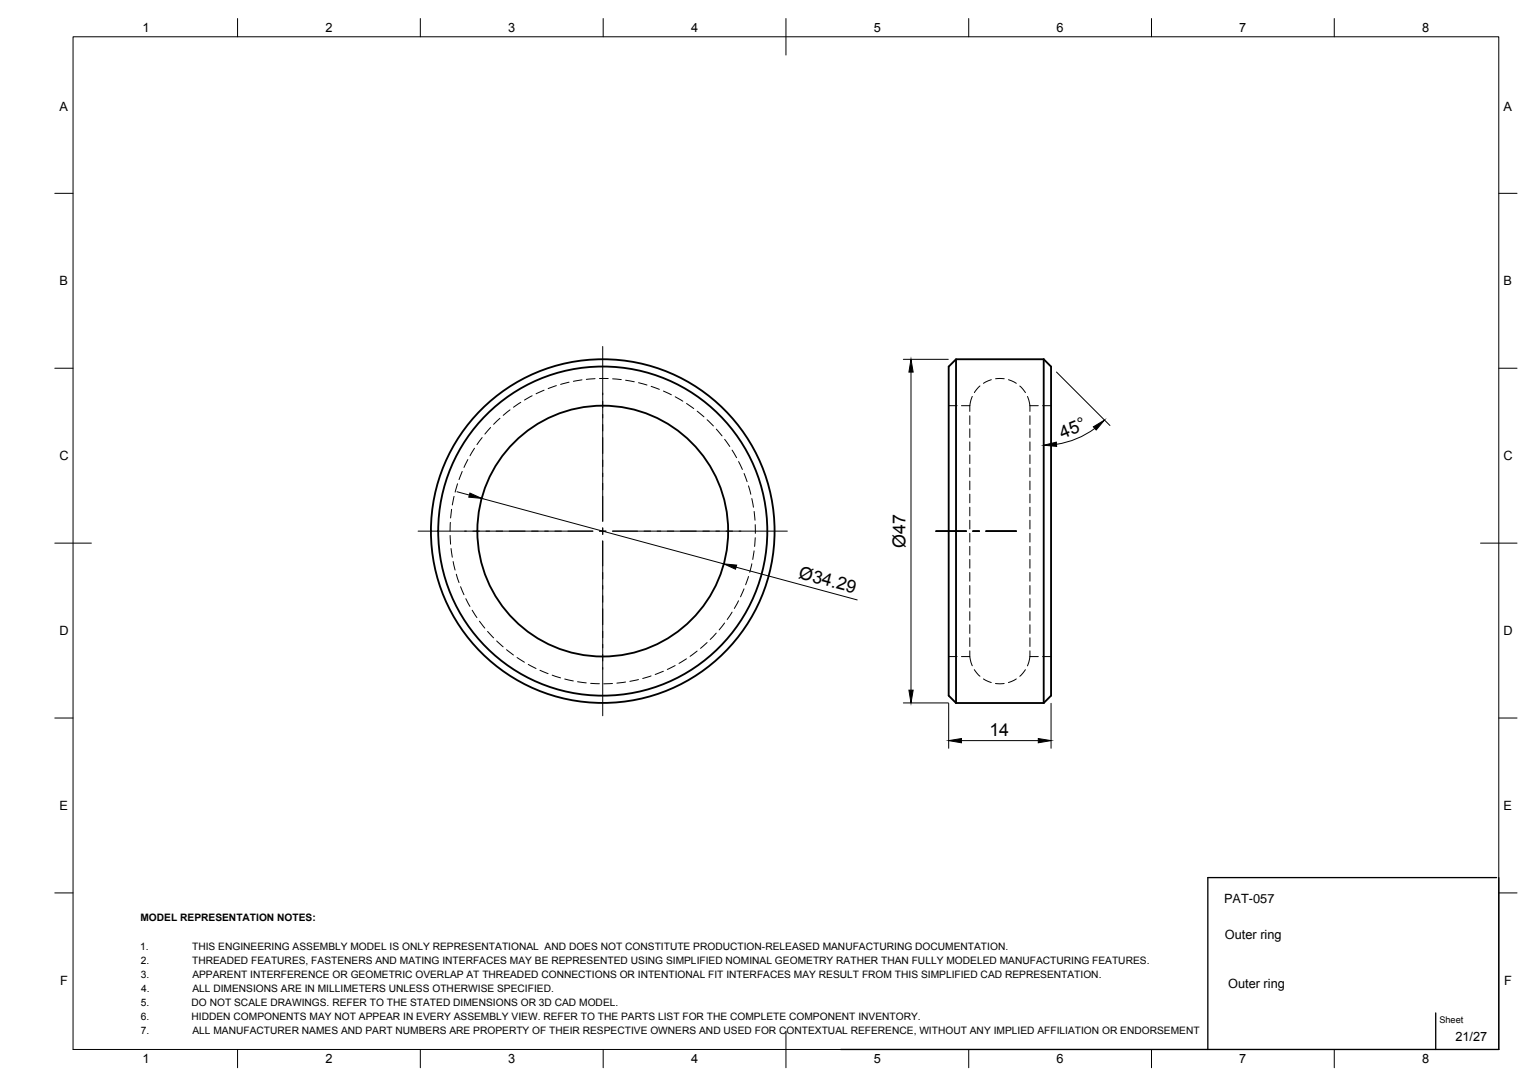
ISO-10303-21;
HEADER;
/* Generated by software containing ST-Developer
 * from STEP Tools, Inc. (www.steptools.com) 
 */

FILE_DESCRIPTION(
/* description */ ('Bearing-mounted hook block'),
/* implementation_level */ '2;1');

FILE_NAME(
/* name */ 'Outer ring.step',
/* time_stamp */ '2026-10-28T22:30:11-07:00',
/* author */ (''),
/* organization */ (''),
/* preprocessor_version */ 'ST-DEVELOPER v20.2',
/* originating_system */ 'Autodesk Translation Framework v15.17.0.0',
/* authorisation */ '');

FILE_SCHEMA (('AUTOMOTIVE_DESIGN { 1 0 10303 214 3 1 1 }'));
ENDSEC;

DATA;
#10=MECHANICAL_DESIGN_GEOMETRIC_PRESENTATION_REPRESENTATION('',(#338),#7609);
#46=TOROIDAL_SURFACE('',#4525,1.675,0.412776);
#264=CONICAL_SURFACE('',#4536,2.3,0.785398163397449);
#265=CONICAL_SURFACE('',#4540,2.3,0.785398163397449);
#290=SHAPE_REPRESENTATION_RELATIONSHIP('SRR','None',#7739,#314);
#314=ADVANCED_BREP_SHAPE_REPRESENTATION('',(#368),#7599);
#338=STYLED_ITEM('',(#7931),#368);
#368=MANIFOLD_SOLID_BREP('Body1',#3936);
#530=LINE('',#6748,#760);
#531=LINE('',#6757,#761);
#532=LINE('',#6761,#762);
#533=LINE('',#6765,#763);
#534=LINE('',#6768,#764);
#760=VECTOR('',#5531,1.71469);
#761=VECTOR('',#5542,2.3);
#762=VECTOR('',#5547,2.35);
#763=VECTOR('',#5552,2.3);
#764=VECTOR('',#5557,1.71469);
#895=CYLINDRICAL_SURFACE('',#4531,1.71469);
#896=CYLINDRICAL_SURFACE('',#4538,2.35);
#897=CYLINDRICAL_SURFACE('',#4543,1.71469);
#976=FACE_BOUND('',#1433,.T.);
#977=FACE_BOUND('',#1438,.T.);
#1139=FACE_OUTER_BOUND('',#1430,.T.);
#1140=FACE_OUTER_BOUND('',#1431,.T.);
#1141=FACE_OUTER_BOUND('',#1432,.T.);
#1142=FACE_OUTER_BOUND('',#1434,.T.);
#1143=FACE_OUTER_BOUND('',#1435,.T.);
#1144=FACE_OUTER_BOUND('',#1436,.T.);
#1145=FACE_OUTER_BOUND('',#1437,.T.);
#1146=FACE_OUTER_BOUND('',#1439,.T.);
#1430=EDGE_LOOP('',(#3156,#3157,#3158,#3159,#3160,#3161));
#1431=EDGE_LOOP('',(#3162,#3163,#3164,#3165,#3166));
#1432=EDGE_LOOP('',(#3167));
#1433=EDGE_LOOP('',(#3168));
#1434=EDGE_LOOP('',(#3169,#3170,#3171,#3172));
#1435=EDGE_LOOP('',(#3173,#3174,#3175,#3176));
#1436=EDGE_LOOP('',(#3177,#3178,#3179,#3180));
#1437=EDGE_LOOP('',(#3181));
#1438=EDGE_LOOP('',(#3182));
#1439=EDGE_LOOP('',(#3183,#3184,#3185,#3186,#3187));
#1678=CIRCLE('',#4526,1.71469);
#1679=CIRCLE('',#4527,1.71469);
#1680=CIRCLE('',#4528,0.412776);
#1681=CIRCLE('',#4529,1.71469);
#1682=CIRCLE('',#4530,1.71469);
#1683=CIRCLE('',#4532,1.71469);
#1684=CIRCLE('',#4534,2.25);
#1685=CIRCLE('',#4535,1.71469);
#1686=CIRCLE('',#4537,2.35);
#1687=CIRCLE('',#4539,2.35);
#1688=CIRCLE('',#4541,2.25);
#1962=VERTEX_POINT('',#6736);
#1963=VERTEX_POINT('',#6737);
#1964=VERTEX_POINT('',#6740);
#1965=VERTEX_POINT('',#6742);
#1966=VERTEX_POINT('',#6746);
#1967=VERTEX_POINT('',#6750);
#1968=VERTEX_POINT('',#6752);
#1969=VERTEX_POINT('',#6755);
#1970=VERTEX_POINT('',#6759);
#1971=VERTEX_POINT('',#6763);
#2388=EDGE_CURVE('',#1962,#1963,#1678,.T.);
#2389=EDGE_CURVE('',#1963,#1962,#1679,.T.);
#2390=EDGE_CURVE('',#1963,#1964,#1680,.T.);
#2391=EDGE_CURVE('',#1965,#1964,#1681,.T.);
#2392=EDGE_CURVE('',#1964,#1965,#1682,.T.);
#2393=EDGE_CURVE('',#1966,#1966,#1683,.T.);
#2394=EDGE_CURVE('',#1966,#1965,#530,.T.);
#2395=EDGE_CURVE('',#1967,#1967,#1684,.T.);
#2396=EDGE_CURVE('',#1968,#1968,#1685,.T.);
#2397=EDGE_CURVE('',#1969,#1969,#1686,.T.);
#2398=EDGE_CURVE('',#1969,#1967,#531,.T.);
#2399=EDGE_CURVE('',#1970,#1970,#1687,.T.);
#2400=EDGE_CURVE('',#1970,#1969,#532,.T.);
#2401=EDGE_CURVE('',#1971,#1971,#1688,.T.);
#2402=EDGE_CURVE('',#1971,#1970,#533,.T.);
#2403=EDGE_CURVE('',#1962,#1968,#534,.T.);
#3156=ORIENTED_EDGE('',*,*,#2388,.F.);
#3157=ORIENTED_EDGE('',*,*,#2389,.F.);
#3158=ORIENTED_EDGE('',*,*,#2390,.T.);
#3159=ORIENTED_EDGE('',*,*,#2391,.F.);
#3160=ORIENTED_EDGE('',*,*,#2392,.F.);
#3161=ORIENTED_EDGE('',*,*,#2390,.F.);
#3162=ORIENTED_EDGE('',*,*,#2393,.T.);
#3163=ORIENTED_EDGE('',*,*,#2394,.T.);
#3164=ORIENTED_EDGE('',*,*,#2391,.T.);
#3165=ORIENTED_EDGE('',*,*,#2392,.T.);
#3166=ORIENTED_EDGE('',*,*,#2394,.F.);
#3167=ORIENTED_EDGE('',*,*,#2395,.F.);
#3168=ORIENTED_EDGE('',*,*,#2396,.T.);
#3169=ORIENTED_EDGE('',*,*,#2397,.F.);
#3170=ORIENTED_EDGE('',*,*,#2398,.T.);
#3171=ORIENTED_EDGE('',*,*,#2395,.T.);
#3172=ORIENTED_EDGE('',*,*,#2398,.F.);
#3173=ORIENTED_EDGE('',*,*,#2399,.F.);
#3174=ORIENTED_EDGE('',*,*,#2400,.T.);
#3175=ORIENTED_EDGE('',*,*,#2397,.T.);
#3176=ORIENTED_EDGE('',*,*,#2400,.F.);
#3177=ORIENTED_EDGE('',*,*,#2401,.F.);
#3178=ORIENTED_EDGE('',*,*,#2402,.T.);
#3179=ORIENTED_EDGE('',*,*,#2399,.T.);
#3180=ORIENTED_EDGE('',*,*,#2402,.F.);
#3181=ORIENTED_EDGE('',*,*,#2401,.T.);
#3182=ORIENTED_EDGE('',*,*,#2393,.F.);
#3183=ORIENTED_EDGE('',*,*,#2388,.T.);
#3184=ORIENTED_EDGE('',*,*,#2389,.T.);
#3185=ORIENTED_EDGE('',*,*,#2403,.T.);
#3186=ORIENTED_EDGE('',*,*,#2396,.F.);
#3187=ORIENTED_EDGE('',*,*,#2403,.F.);
#3633=PLANE('',#4533);
#3634=PLANE('',#4542);
#3821=ADVANCED_FACE('',(#1139),#46,.F.);
#3822=ADVANCED_FACE('',(#1140),#895,.F.);
#3823=ADVANCED_FACE('',(#1141,#976),#3633,.T.);
#3824=ADVANCED_FACE('',(#1142),#264,.T.);
#3825=ADVANCED_FACE('',(#1143),#896,.T.);
#3826=ADVANCED_FACE('',(#1144),#265,.T.);
#3827=ADVANCED_FACE('',(#1145,#977),#3634,.T.);
#3828=ADVANCED_FACE('',(#1146),#897,.F.);
#3936=CLOSED_SHELL('',(#3821,#3822,#3823,#3824,#3825,#3826,#3827,#3828));
#4524=AXIS2_PLACEMENT_3D('',#6734,#5513,#5514);
#4525=AXIS2_PLACEMENT_3D('',#6735,#5515,#5516);
#4526=AXIS2_PLACEMENT_3D('',#6738,#5517,#5518);
#4527=AXIS2_PLACEMENT_3D('',#6739,#5519,#5520);
#4528=AXIS2_PLACEMENT_3D('',#6741,#5521,#5522);
#4529=AXIS2_PLACEMENT_3D('',#6743,#5523,#5524);
#4530=AXIS2_PLACEMENT_3D('',#6744,#5525,#5526);
#4531=AXIS2_PLACEMENT_3D('',#6745,#5527,#5528);
#4532=AXIS2_PLACEMENT_3D('',#6747,#5529,#5530);
#4533=AXIS2_PLACEMENT_3D('',#6749,#5532,#5533);
#4534=AXIS2_PLACEMENT_3D('',#6751,#5534,#5535);
#4535=AXIS2_PLACEMENT_3D('',#6753,#5536,#5537);
#4536=AXIS2_PLACEMENT_3D('',#6754,#5538,#5539);
#4537=AXIS2_PLACEMENT_3D('',#6756,#5540,#5541);
#4538=AXIS2_PLACEMENT_3D('',#6758,#5543,#5544);
#4539=AXIS2_PLACEMENT_3D('',#6760,#5545,#5546);
#4540=AXIS2_PLACEMENT_3D('',#6762,#5548,#5549);
#4541=AXIS2_PLACEMENT_3D('',#6764,#5550,#5551);
#4542=AXIS2_PLACEMENT_3D('',#6766,#5553,#5554);
#4543=AXIS2_PLACEMENT_3D('',#6767,#5555,#5556);
#5513=DIRECTION('axis',(0.,0.,1.));
#5514=DIRECTION('refdir',(1.,0.,0.));
#5515=DIRECTION('center_axis',(0.,-1.,0.));
#5516=DIRECTION('ref_axis',(0.,0.,-1.));
#5517=DIRECTION('center_axis',(0.,-1.,0.));
#5518=DIRECTION('ref_axis',(1.,0.,0.));
#5519=DIRECTION('center_axis',(0.,-1.,0.));
#5520=DIRECTION('ref_axis',(1.,0.,0.));
#5521=DIRECTION('center_axis',(1.,0.,1.22464679914735E-16));
#5522=DIRECTION('ref_axis',(-1.22464679914735E-16,0.,1.));
#5523=DIRECTION('center_axis',(0.,1.,0.));
#5524=DIRECTION('ref_axis',(1.,0.,0.));
#5525=DIRECTION('center_axis',(0.,1.,0.));
#5526=DIRECTION('ref_axis',(1.,0.,0.));
#5527=DIRECTION('center_axis',(0.,-1.,0.));
#5528=DIRECTION('ref_axis',(1.,0.,0.));
#5529=DIRECTION('center_axis',(0.,-1.,0.));
#5530=DIRECTION('ref_axis',(1.,0.,0.));
#5531=DIRECTION('',(0.,1.,0.));
#5532=DIRECTION('center_axis',(0.,1.,0.));
#5533=DIRECTION('ref_axis',(0.,0.,1.));
#5534=DIRECTION('center_axis',(0.,-1.,0.));
#5535=DIRECTION('ref_axis',(1.,0.,0.));
#5536=DIRECTION('center_axis',(0.,-1.,0.));
#5537=DIRECTION('ref_axis',(1.,0.,0.));
#5538=DIRECTION('center_axis',(0.,-1.,0.));
#5539=DIRECTION('ref_axis',(1.,0.,0.));
#5540=DIRECTION('center_axis',(0.,-1.,0.));
#5541=DIRECTION('ref_axis',(1.,0.,0.));
#5542=DIRECTION('',(0.707106781186548,0.707106781186547,8.65956056235494E-17));
#5543=DIRECTION('center_axis',(0.,-1.,0.));
#5544=DIRECTION('ref_axis',(1.,0.,0.));
#5545=DIRECTION('center_axis',(0.,-1.,0.));
#5546=DIRECTION('ref_axis',(1.,0.,0.));
#5547=DIRECTION('',(0.,1.,0.));
#5548=DIRECTION('center_axis',(0.,1.,0.));
#5549=DIRECTION('ref_axis',(1.,0.,0.));
#5550=DIRECTION('center_axis',(0.,-1.,0.));
#5551=DIRECTION('ref_axis',(1.,0.,0.));
#5552=DIRECTION('',(-0.707106781186548,0.707106781186547,-8.65956056235494E-17));
#5553=DIRECTION('center_axis',(0.,-1.,0.));
#5554=DIRECTION('ref_axis',(0.,0.,-1.));
#5555=DIRECTION('center_axis',(0.,-1.,0.));
#5556=DIRECTION('ref_axis',(1.,0.,0.));
#5557=DIRECTION('',(0.,1.,0.));
#6734=CARTESIAN_POINT('',(0.,0.,0.));
#6735=CARTESIAN_POINT('Origin',(0.,0.,0.));
#6736=CARTESIAN_POINT('',(-1.71469,0.410863395882378,-2.09988962002998E-16));
#6737=CARTESIAN_POINT('',(-2.09988962002998E-16,0.410863395882378,1.71469));
#6738=CARTESIAN_POINT('Origin',(0.,0.410863395882378,0.));
#6739=CARTESIAN_POINT('Origin',(0.,0.410863395882378,0.));
#6740=CARTESIAN_POINT('',(-2.09988962002998E-16,-0.410863395882378,1.71469));
#6741=CARTESIAN_POINT('Origin',(-2.05128338857182E-16,0.,1.675));
#6742=CARTESIAN_POINT('',(-1.71469,-0.410863395882378,2.09988962002998E-16));
#6743=CARTESIAN_POINT('Origin',(0.,-0.410863395882378,0.));
#6744=CARTESIAN_POINT('Origin',(0.,-0.410863395882378,0.));
#6745=CARTESIAN_POINT('Origin',(0.,0.,0.));
#6746=CARTESIAN_POINT('',(-1.71469,-0.7,-2.09988962002998E-16));
#6747=CARTESIAN_POINT('Origin',(0.,-0.7,0.));
#6748=CARTESIAN_POINT('',(-1.71469,0.,-2.09988962002998E-16));
#6749=CARTESIAN_POINT('Origin',(2.25,0.7,0.));
#6750=CARTESIAN_POINT('',(-2.25,0.7,-2.75545529808154E-16));
#6751=CARTESIAN_POINT('Origin',(0.,0.7,0.));
#6752=CARTESIAN_POINT('',(-1.71469,0.7,-2.09988962002998E-16));
#6753=CARTESIAN_POINT('Origin',(0.,0.7,0.));
#6754=CARTESIAN_POINT('Origin',(0.,0.65,0.));
#6755=CARTESIAN_POINT('',(-2.35,0.6,-2.87791997799628E-16));
#6756=CARTESIAN_POINT('Origin',(0.,0.6,0.));
#6757=CARTESIAN_POINT('',(-2.3,0.65,-2.81668763803891E-16));
#6758=CARTESIAN_POINT('Origin',(0.,0.,0.));
#6759=CARTESIAN_POINT('',(-2.35,-0.6,-2.87791997799628E-16));
#6760=CARTESIAN_POINT('Origin',(0.,-0.6,0.));
#6761=CARTESIAN_POINT('',(-2.35,0.,-2.87791997799628E-16));
#6762=CARTESIAN_POINT('Origin',(0.,-0.65,0.));
#6763=CARTESIAN_POINT('',(-2.25,-0.7,-2.75545529808154E-16));
#6764=CARTESIAN_POINT('Origin',(0.,-0.7,0.));
#6765=CARTESIAN_POINT('',(-2.3,-0.65,-2.81668763803891E-16));
#6766=CARTESIAN_POINT('Origin',(1.71469,-0.7,0.));
#6767=CARTESIAN_POINT('Origin',(0.,0.,0.));
#6768=CARTESIAN_POINT('',(-1.71469,0.,-2.09988962002998E-16));
#7569=UNCERTAINTY_MEASURE_WITH_UNIT(LENGTH_MEASURE(0.001),#7610,
'DISTANCE_ACCURACY_VALUE',
'Maximum model space distance between geometric entities at asserted c
onnectivities');
#7579=UNCERTAINTY_MEASURE_WITH_UNIT(LENGTH_MEASURE(0.001),#7610,
'DISTANCE_ACCURACY_VALUE',
'Maximum model space distance between geometric entities at asserted c
onnectivities');
#7599=(
GEOMETRIC_REPRESENTATION_CONTEXT(3)
GLOBAL_UNCERTAINTY_ASSIGNED_CONTEXT((#7569))
GLOBAL_UNIT_ASSIGNED_CONTEXT((#7610,#7612,#7613))
REPRESENTATION_CONTEXT('','3D')
);
#7609=(
GEOMETRIC_REPRESENTATION_CONTEXT(3)
GLOBAL_UNCERTAINTY_ASSIGNED_CONTEXT((#7579))
GLOBAL_UNIT_ASSIGNED_CONTEXT((#7610,#7612,#7613))
REPRESENTATION_CONTEXT('','3D')
);
#7610=(
LENGTH_UNIT()
NAMED_UNIT(*)
SI_UNIT(.CENTI.,.METRE.)
);
#7612=(
NAMED_UNIT(*)
PLANE_ANGLE_UNIT()
SI_UNIT($,.RADIAN.)
);
#7613=(
NAMED_UNIT(*)
SI_UNIT($,.STERADIAN.)
SOLID_ANGLE_UNIT()
);
#7633=SHAPE_DEFINITION_REPRESENTATION(#7685,#7739);
#7685=PRODUCT_DEFINITION_SHAPE('',$,#7769);
#7739=SHAPE_REPRESENTATION('',(#4524),#7599);
#7749=PRODUCT_DEFINITION_CONTEXT('part definition',#7838,'design');
#7769=PRODUCT_DEFINITION('Outer ring','Outer ring',#7798,#7749);
#7798=PRODUCT_DEFINITION_FORMATION('',$,#7859);
#7838=APPLICATION_CONTEXT(
'Core Data for Automotive Mechanical Design Process');
#7839=PRODUCT_CONTEXT('part definition',#7838,'mechanical');
#7859=PRODUCT('Outer ring','Outer ring','Outer ring',(#7839));
#7925=COLOUR_RGB('Grey',0.48,0.52,0.57);
#7926=FILL_AREA_STYLE_COLOUR('',#7925);
#7927=FILL_AREA_STYLE('',(#7926));
#7928=SURFACE_STYLE_FILL_AREA(#7927);
#7929=SURFACE_SIDE_STYLE('',(#7928));
#7930=SURFACE_STYLE_USAGE(.BOTH.,#7929);
#7931=PRESENTATION_STYLE_ASSIGNMENT((#7930));
ENDSEC;
END-ISO-10303-21;
